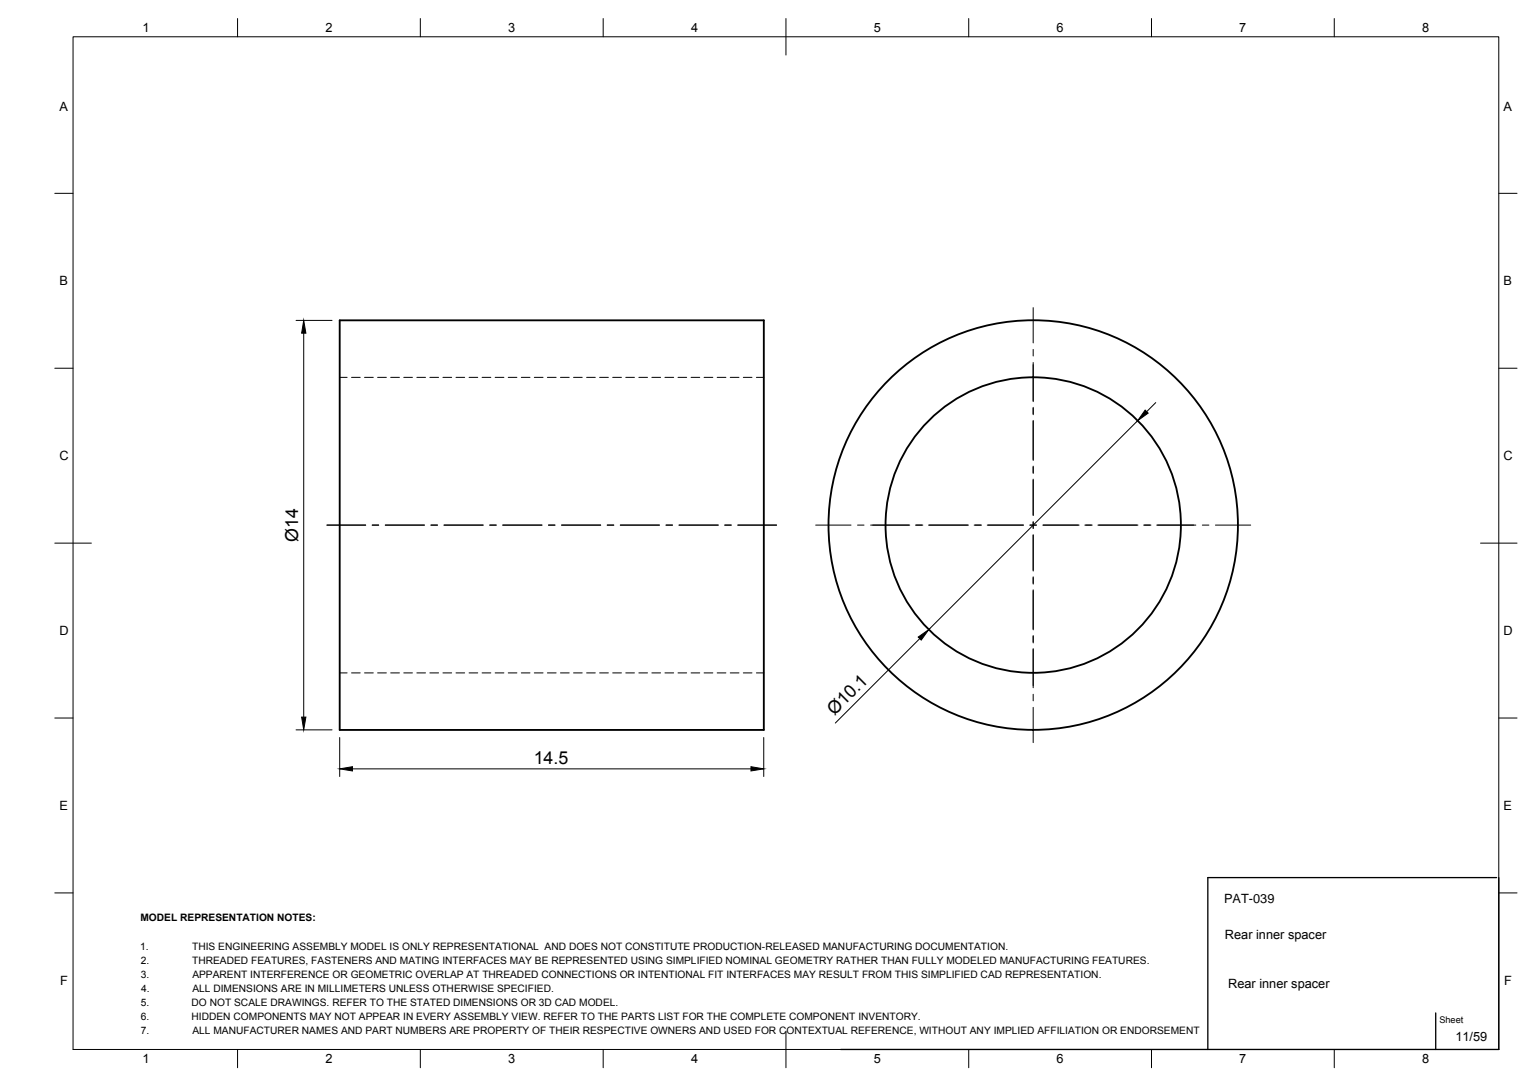
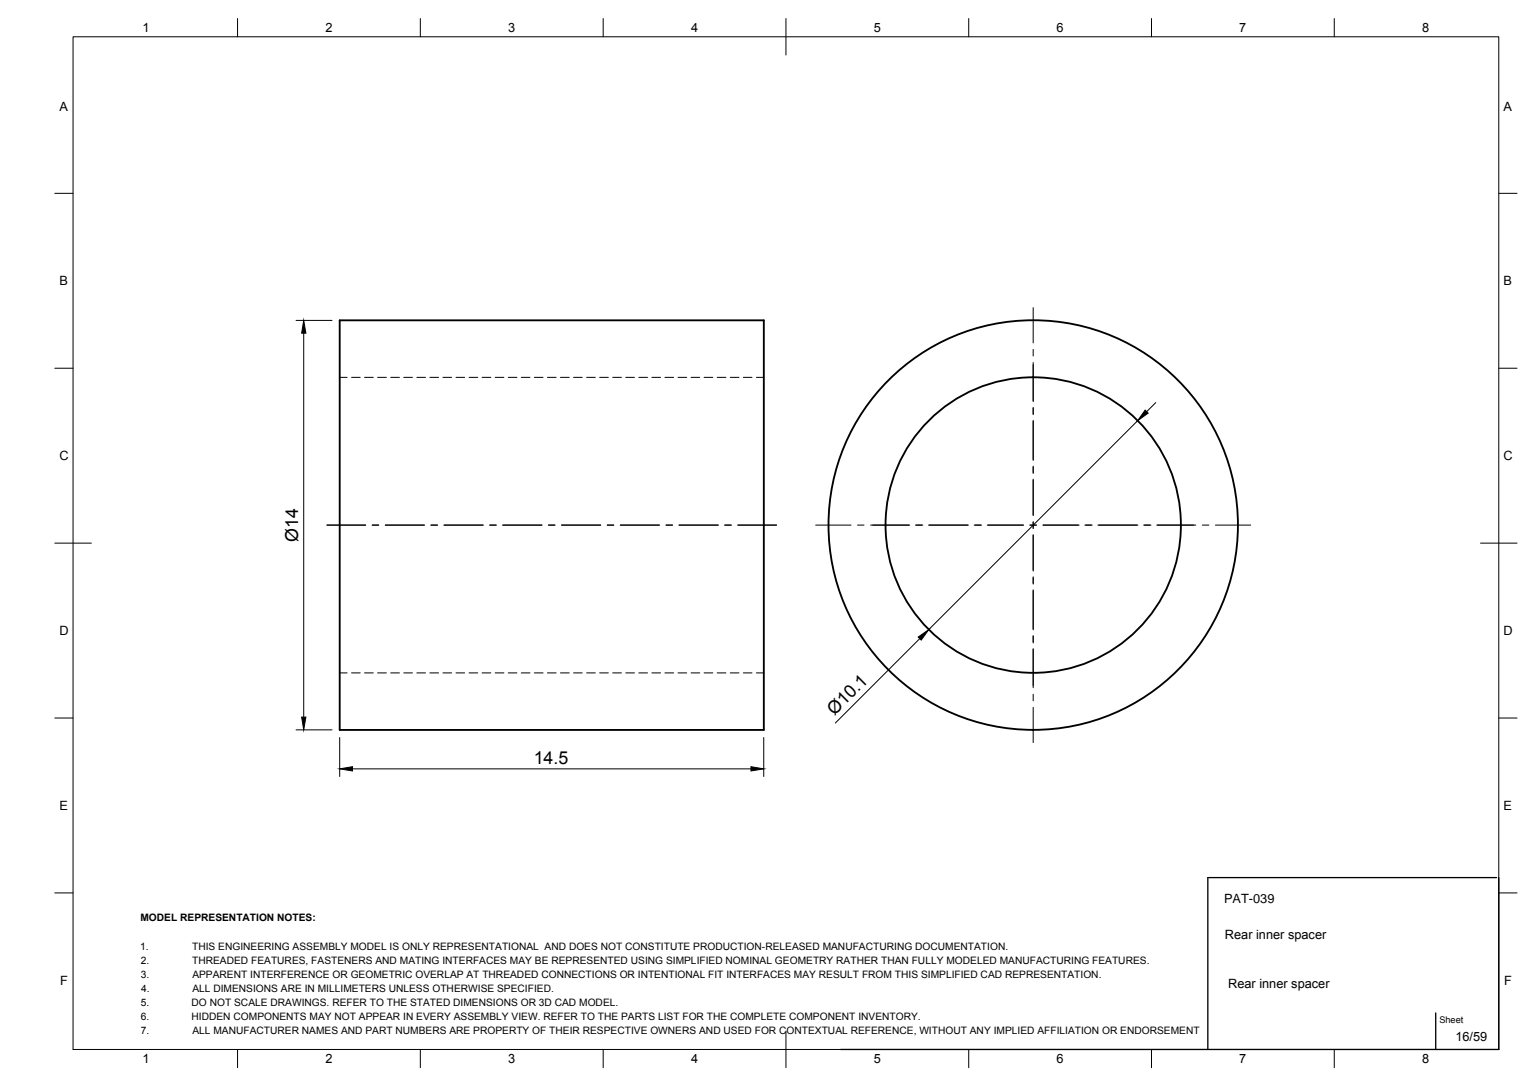
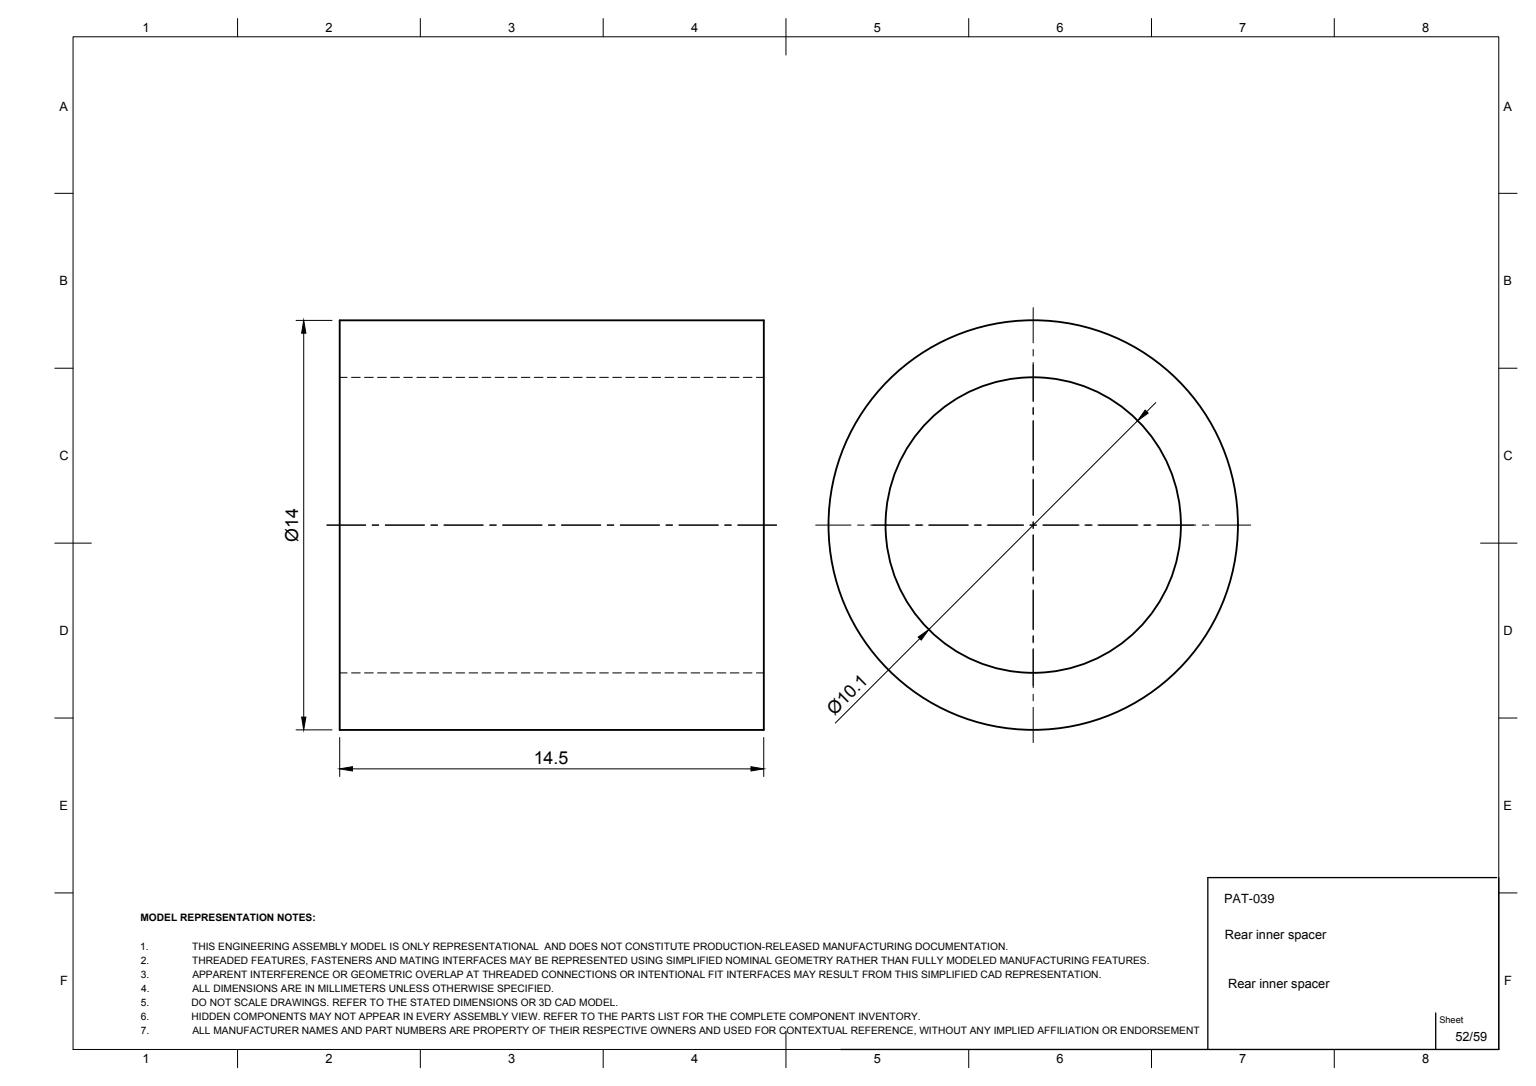
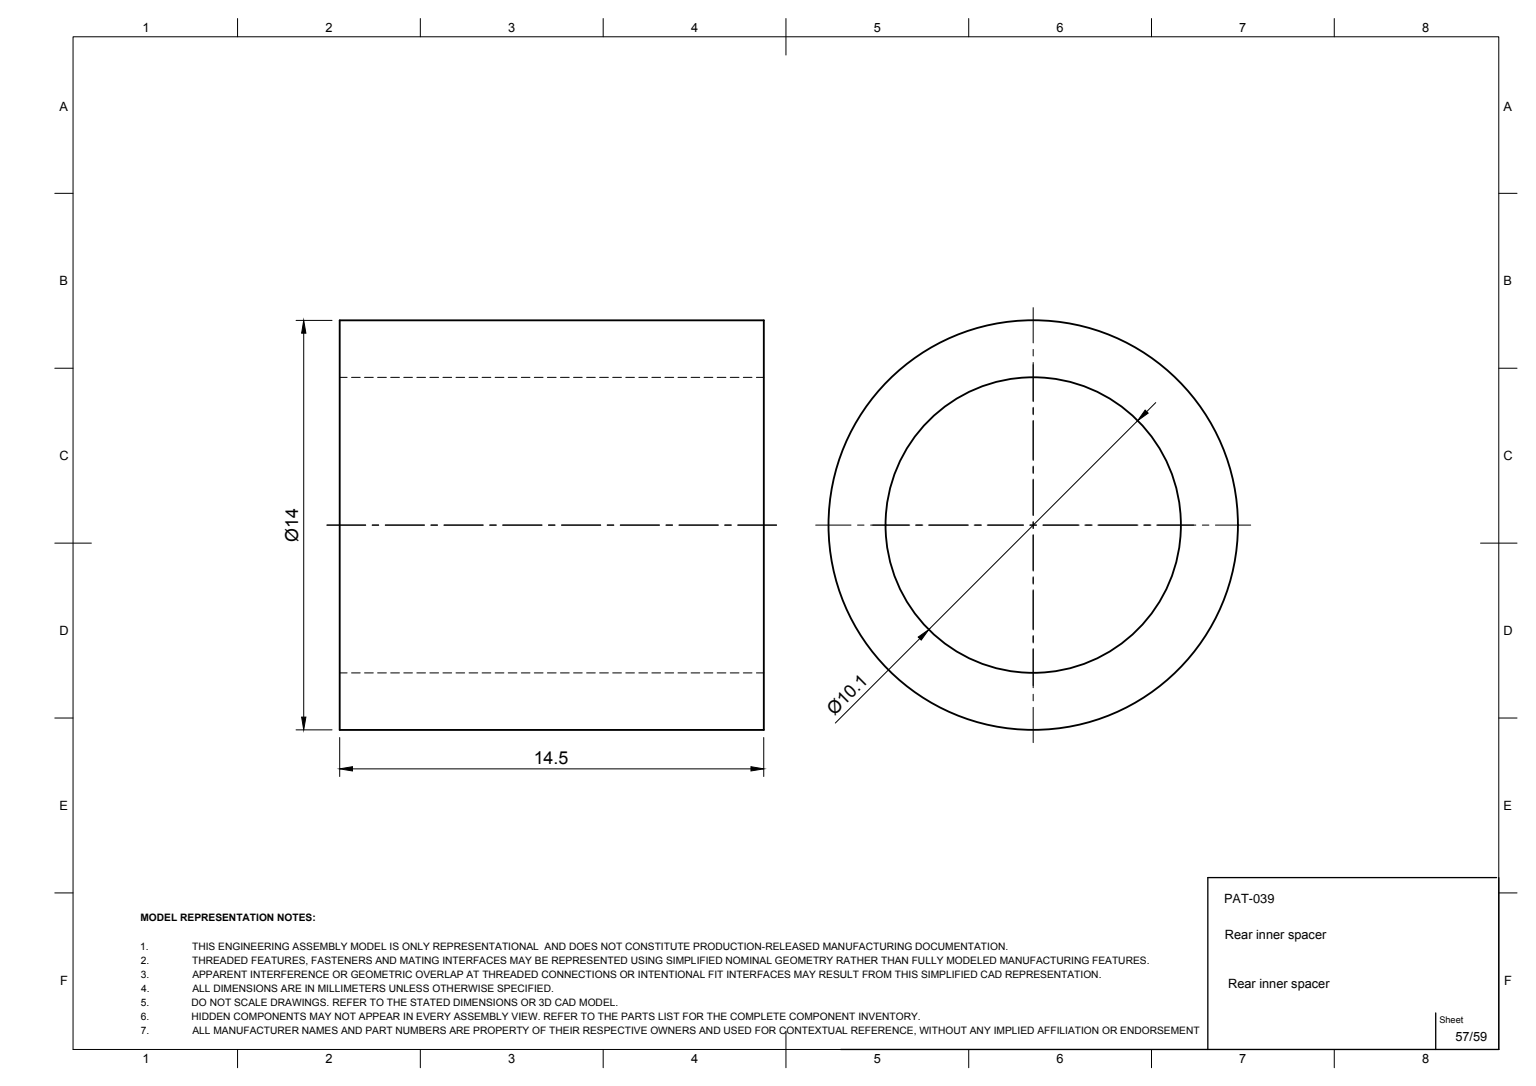
ISO-10303-21;
HEADER;
/* Generated by software containing ST-Developer
 * from STEP Tools, Inc. (www.steptools.com) 
 */

FILE_DESCRIPTION(
/* description */ ('Four-bar parallelogram arm'),
/* implementation_level */ '2;1');

FILE_NAME(
/* name */ 'Rear inner spacer.step',
/* time_stamp */ '2026-10-28T03:24:55-07:00',
/* author */ (''),
/* organization */ (''),
/* preprocessor_version */ 'ST-DEVELOPER v20.2',
/* originating_system */ 'Autodesk Translation Framework v15.17.0.0',
/* authorisation */ '');

FILE_SCHEMA (('AUTOMOTIVE_DESIGN { 1 0 10303 214 3 1 1 }'));
ENDSEC;

DATA;
#10=MECHANICAL_DESIGN_GEOMETRIC_PRESENTATION_REPRESENTATION('',(#628),#14512);
#528=SHAPE_REPRESENTATION_RELATIONSHIP('SRR','None',#14749,#578);
#578=ADVANCED_BREP_SHAPE_REPRESENTATION('',(#686),#14464);
#628=STYLED_ITEM('',(#15080),#686);
#686=MANIFOLD_SOLID_BREP('Body1',#7332);
#779=FACE_BOUND('',#1730,.T.);
#780=FACE_BOUND('',#1732,.T.);
#1042=PLANE('',#8067);
#1043=PLANE('',#8068);
#1263=FACE_OUTER_BOUND('',#1727,.T.);
#1264=FACE_OUTER_BOUND('',#1728,.T.);
#1265=FACE_OUTER_BOUND('',#1729,.T.);
#1266=FACE_OUTER_BOUND('',#1731,.T.);
#1727=EDGE_LOOP('',(#5264,#5265,#5266,#5267));
#1728=EDGE_LOOP('',(#5268,#5269,#5270,#5271));
#1729=EDGE_LOOP('',(#5272));
#1730=EDGE_LOOP('',(#5273));
#1731=EDGE_LOOP('',(#5274));
#1732=EDGE_LOOP('',(#5275));
#2398=LINE('',#11733,#2792);
#2399=LINE('',#11739,#2793);
#2792=VECTOR('',#9306,0.505);
#2793=VECTOR('',#9313,0.7);
#3152=CIRCLE('',#8062,0.505);
#3153=CIRCLE('',#8063,0.505);
#3154=CIRCLE('',#8065,0.7);
#3155=CIRCLE('',#8066,0.7);
#3637=VERTEX_POINT('',#11730);
#3638=VERTEX_POINT('',#11732);
#3639=VERTEX_POINT('',#11736);
#3640=VERTEX_POINT('',#11738);
#4263=EDGE_CURVE('',#3637,#3637,#3152,.T.);
#4264=EDGE_CURVE('',#3637,#3638,#2398,.T.);
#4265=EDGE_CURVE('',#3638,#3638,#3153,.T.);
#4266=EDGE_CURVE('',#3639,#3639,#3154,.T.);
#4267=EDGE_CURVE('',#3639,#3640,#2399,.T.);
#4268=EDGE_CURVE('',#3640,#3640,#3155,.T.);
#5264=ORIENTED_EDGE('',*,*,#4263,.F.);
#5265=ORIENTED_EDGE('',*,*,#4264,.T.);
#5266=ORIENTED_EDGE('',*,*,#4265,.T.);
#5267=ORIENTED_EDGE('',*,*,#4264,.F.);
#5268=ORIENTED_EDGE('',*,*,#4266,.F.);
#5269=ORIENTED_EDGE('',*,*,#4267,.T.);
#5270=ORIENTED_EDGE('',*,*,#4268,.T.);
#5271=ORIENTED_EDGE('',*,*,#4267,.F.);
#5272=ORIENTED_EDGE('',*,*,#4266,.T.);
#5273=ORIENTED_EDGE('',*,*,#4263,.T.);
#5274=ORIENTED_EDGE('',*,*,#4268,.F.);
#5275=ORIENTED_EDGE('',*,*,#4265,.F.);
#6740=CYLINDRICAL_SURFACE('',#8061,0.505);
#6741=CYLINDRICAL_SURFACE('',#8064,0.7);
#6968=ADVANCED_FACE('',(#1263),#6740,.F.);
#6969=ADVANCED_FACE('',(#1264),#6741,.T.);
#6970=ADVANCED_FACE('',(#1265,#779),#1042,.T.);
#6971=ADVANCED_FACE('',(#1266,#780),#1043,.F.);
#7332=CLOSED_SHELL('',(#6968,#6969,#6970,#6971));
#8060=AXIS2_PLACEMENT_3D('',#11728,#9300,#9301);
#8061=AXIS2_PLACEMENT_3D('',#11729,#9302,#9303);
#8062=AXIS2_PLACEMENT_3D('',#11731,#9304,#9305);
#8063=AXIS2_PLACEMENT_3D('',#11734,#9307,#9308);
#8064=AXIS2_PLACEMENT_3D('',#11735,#9309,#9310);
#8065=AXIS2_PLACEMENT_3D('',#11737,#9311,#9312);
#8066=AXIS2_PLACEMENT_3D('',#11740,#9314,#9315);
#8067=AXIS2_PLACEMENT_3D('',#11741,#9316,#9317);
#8068=AXIS2_PLACEMENT_3D('',#11742,#9318,#9319);
#9300=DIRECTION('axis',(0.,0.,1.));
#9301=DIRECTION('refdir',(1.,0.,0.));
#9302=DIRECTION('center_axis',(0.,1.,0.));
#9303=DIRECTION('ref_axis',(1.,0.,0.));
#9304=DIRECTION('center_axis',(0.,-1.,0.));
#9305=DIRECTION('ref_axis',(1.,0.,0.));
#9306=DIRECTION('',(0.,-1.,0.));
#9307=DIRECTION('center_axis',(0.,-1.,0.));
#9308=DIRECTION('ref_axis',(1.,0.,0.));
#9309=DIRECTION('center_axis',(0.,1.,0.));
#9310=DIRECTION('ref_axis',(1.,0.,0.));
#9311=DIRECTION('center_axis',(0.,1.,0.));
#9312=DIRECTION('ref_axis',(1.,0.,0.));
#9313=DIRECTION('',(0.,-1.,0.));
#9314=DIRECTION('center_axis',(0.,1.,0.));
#9315=DIRECTION('ref_axis',(1.,0.,0.));
#9316=DIRECTION('center_axis',(0.,1.,0.));
#9317=DIRECTION('ref_axis',(1.,0.,0.));
#9318=DIRECTION('center_axis',(0.,1.,0.));
#9319=DIRECTION('ref_axis',(1.,0.,0.));
#11728=CARTESIAN_POINT('',(0.,0.,0.));
#11729=CARTESIAN_POINT('Origin',(0.,1.05,8.));
#11730=CARTESIAN_POINT('',(-0.505,2.5,8.));
#11731=CARTESIAN_POINT('Origin',(0.,2.5,8.));
#11732=CARTESIAN_POINT('',(-0.505,1.05,8.));
#11733=CARTESIAN_POINT('',(-0.505,1.05,8.));
#11734=CARTESIAN_POINT('Origin',(0.,1.05,8.));
#11735=CARTESIAN_POINT('Origin',(0.,1.05,8.));
#11736=CARTESIAN_POINT('',(-0.7,2.5,8.));
#11737=CARTESIAN_POINT('Origin',(0.,2.5,8.));
#11738=CARTESIAN_POINT('',(-0.7,1.05,8.));
#11739=CARTESIAN_POINT('',(-0.7,1.05,8.));
#11740=CARTESIAN_POINT('Origin',(0.,1.05,8.));
#11741=CARTESIAN_POINT('Origin',(0.,2.5,8.));
#11742=CARTESIAN_POINT('Origin',(0.,1.05,8.));
#14407=UNCERTAINTY_MEASURE_WITH_UNIT(LENGTH_MEASURE(0.001),#14513,
'DISTANCE_ACCURACY_VALUE',
'Maximum model space distance between geometric entities at asserted c
onnectivities');
#14455=UNCERTAINTY_MEASURE_WITH_UNIT(LENGTH_MEASURE(0.001),#14513,
'DISTANCE_ACCURACY_VALUE',
'Maximum model space distance between geometric entities at asserted c
onnectivities');
#14464=(
GEOMETRIC_REPRESENTATION_CONTEXT(3)
GLOBAL_UNCERTAINTY_ASSIGNED_CONTEXT((#14407))
GLOBAL_UNIT_ASSIGNED_CONTEXT((#14513,#14515,#14516))
REPRESENTATION_CONTEXT('','3D')
);
#14512=(
GEOMETRIC_REPRESENTATION_CONTEXT(3)
GLOBAL_UNCERTAINTY_ASSIGNED_CONTEXT((#14455))
GLOBAL_UNIT_ASSIGNED_CONTEXT((#14513,#14515,#14516))
REPRESENTATION_CONTEXT('','3D')
);
#14513=(
LENGTH_UNIT()
NAMED_UNIT(*)
SI_UNIT(.CENTI.,.METRE.)
);
#14515=(
NAMED_UNIT(*)
PLANE_ANGLE_UNIT()
SI_UNIT($,.RADIAN.)
);
#14516=(
NAMED_UNIT(*)
SI_UNIT($,.STERADIAN.)
SOLID_ANGLE_UNIT()
);
#14525=SHAPE_DEFINITION_REPRESENTATION(#14581,#14749);
#14581=PRODUCT_DEFINITION_SHAPE('',$,#14806);
#14749=SHAPE_REPRESENTATION('',(#8060),#14464);
#14797=PRODUCT_DEFINITION_CONTEXT('part definition',#14967,'design');
#14806=PRODUCT_DEFINITION('Rear inner spacer','Rear inner spacer',#14862,
#14797);
#14862=PRODUCT_DEFINITION_FORMATION('',$,#14977);
#14967=APPLICATION_CONTEXT(
'Core Data for Automotive Mechanical Design Process');
#14968=PRODUCT_CONTEXT('part definition',#14967,'mechanical');
#14977=PRODUCT('Rear inner spacer','Rear inner spacer',
'Rear inner spacer',(#14968));
#15074=COLOUR_RGB('Sky Blue',0.24,0.69,0.87);
#15075=FILL_AREA_STYLE_COLOUR('',#15074);
#15076=FILL_AREA_STYLE('',(#15075));
#15077=SURFACE_STYLE_FILL_AREA(#15076);
#15078=SURFACE_SIDE_STYLE('',(#15077));
#15079=SURFACE_STYLE_USAGE(.BOTH.,#15078);
#15080=PRESENTATION_STYLE_ASSIGNMENT((#15079));
ENDSEC;
END-ISO-10303-21;
